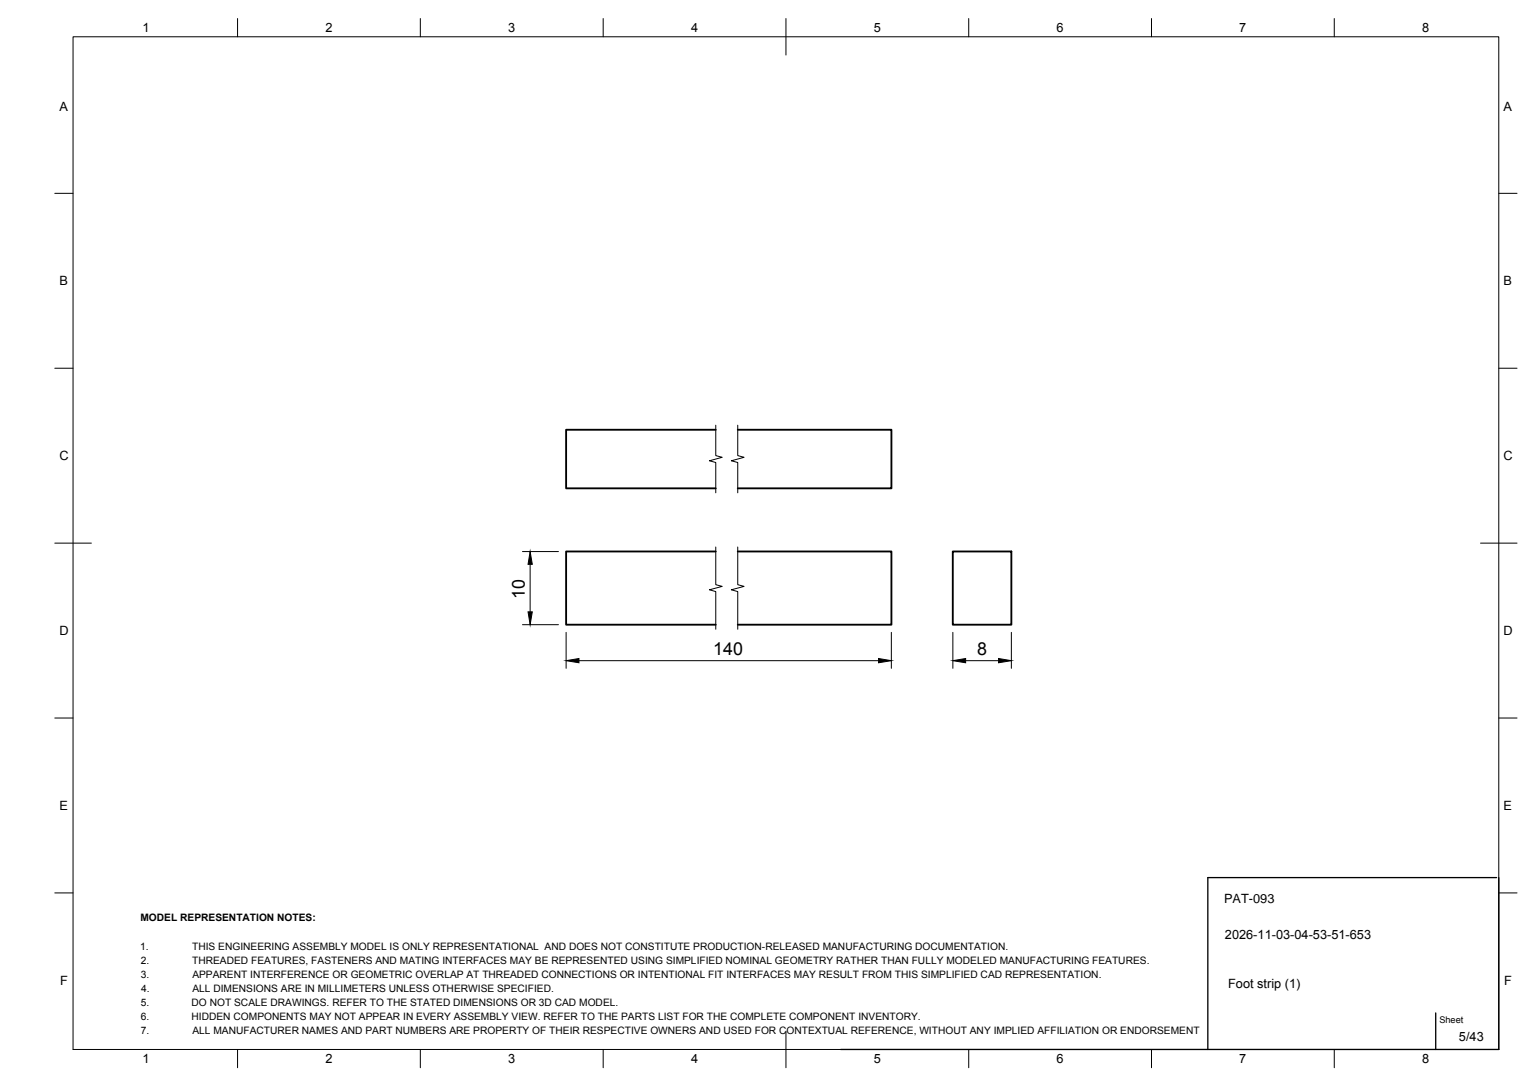
ISO-10303-21;
HEADER;
/* Generated by software containing ST-Developer
 * from STEP Tools, Inc. (www.steptools.com) 
 */

FILE_DESCRIPTION(
/* description */ ('Self-centering screw clamp'),
/* implementation_level */ '2;1');

FILE_NAME(
/* name */ 'Foot strip (1).step',
/* time_stamp */ '2026-10-28T03:25:31-07:00',
/* author */ (''),
/* organization */ (''),
/* preprocessor_version */ 'ST-DEVELOPER v20.2',
/* originating_system */ 'Autodesk Translation Framework v15.17.0.0',
/* authorisation */ '');

FILE_SCHEMA (('AUTOMOTIVE_DESIGN { 1 0 10303 214 3 1 1 }'));
ENDSEC;

DATA;
#10=MECHANICAL_DESIGN_GEOMETRIC_PRESENTATION_REPRESENTATION('',(#626),#16799);
#544=SHAPE_REPRESENTATION_RELATIONSHIP('SRR','None',#17017,#585);
#585=ADVANCED_BREP_SHAPE_REPRESENTATION('',(#674),#16755);
#626=STYLED_ITEM('',(#17312),#674);
#674=MANIFOLD_SOLID_BREP('Body1',#9077);
#1026=PLANE('',#9630);
#1027=PLANE('',#9631);
#1028=PLANE('',#9632);
#1029=PLANE('',#9633);
#1030=PLANE('',#9634);
#1031=PLANE('',#9635);
#1297=FACE_OUTER_BOUND('',#1825,.T.);
#1298=FACE_OUTER_BOUND('',#1826,.T.);
#1299=FACE_OUTER_BOUND('',#1827,.T.);
#1300=FACE_OUTER_BOUND('',#1828,.T.);
#1301=FACE_OUTER_BOUND('',#1829,.T.);
#1302=FACE_OUTER_BOUND('',#1830,.T.);
#1825=EDGE_LOOP('',(#6223,#6224,#6225,#6226));
#1826=EDGE_LOOP('',(#6227,#6228,#6229,#6230));
#1827=EDGE_LOOP('',(#6231,#6232,#6233,#6234));
#1828=EDGE_LOOP('',(#6235,#6236,#6237,#6238));
#1829=EDGE_LOOP('',(#6239,#6240,#6241,#6242));
#1830=EDGE_LOOP('',(#6243,#6244,#6245,#6246));
#2613=LINE('',#13807,#3186);
#2614=LINE('',#13809,#3187);
#2615=LINE('',#13811,#3188);
#2616=LINE('',#13812,#3189);
#2617=LINE('',#13815,#3190);
#2618=LINE('',#13817,#3191);
#2619=LINE('',#13818,#3192);
#2620=LINE('',#13821,#3193);
#2621=LINE('',#13823,#3194);
#2622=LINE('',#13824,#3195);
#2623=LINE('',#13826,#3196);
#2624=LINE('',#13827,#3197);
#3186=VECTOR('',#10896,1.);
#3187=VECTOR('',#10897,1.);
#3188=VECTOR('',#10898,1.);
#3189=VECTOR('',#10899,1.);
#3190=VECTOR('',#10902,1.);
#3191=VECTOR('',#10903,1.);
#3192=VECTOR('',#10904,1.);
#3193=VECTOR('',#10907,1.);
#3194=VECTOR('',#10908,1.);
#3195=VECTOR('',#10909,1.);
#3196=VECTOR('',#10912,1.);
#3197=VECTOR('',#10913,1.);
#4273=VERTEX_POINT('',#13805);
#4274=VERTEX_POINT('',#13806);
#4275=VERTEX_POINT('',#13808);
#4276=VERTEX_POINT('',#13810);
#4277=VERTEX_POINT('',#13814);
#4278=VERTEX_POINT('',#13816);
#4279=VERTEX_POINT('',#13820);
#4280=VERTEX_POINT('',#13822);
#5036=EDGE_CURVE('',#4273,#4274,#2613,.T.);
#5037=EDGE_CURVE('',#4274,#4275,#2614,.T.);
#5038=EDGE_CURVE('',#4276,#4275,#2615,.T.);
#5039=EDGE_CURVE('',#4273,#4276,#2616,.T.);
#5040=EDGE_CURVE('',#4277,#4273,#2617,.T.);
#5041=EDGE_CURVE('',#4278,#4276,#2618,.T.);
#5042=EDGE_CURVE('',#4277,#4278,#2619,.T.);
#5043=EDGE_CURVE('',#4279,#4277,#2620,.T.);
#5044=EDGE_CURVE('',#4280,#4278,#2621,.T.);
#5045=EDGE_CURVE('',#4279,#4280,#2622,.T.);
#5046=EDGE_CURVE('',#4274,#4279,#2623,.T.);
#5047=EDGE_CURVE('',#4275,#4280,#2624,.T.);
#6223=ORIENTED_EDGE('',*,*,#5036,.T.);
#6224=ORIENTED_EDGE('',*,*,#5037,.T.);
#6225=ORIENTED_EDGE('',*,*,#5038,.F.);
#6226=ORIENTED_EDGE('',*,*,#5039,.F.);
#6227=ORIENTED_EDGE('',*,*,#5040,.T.);
#6228=ORIENTED_EDGE('',*,*,#5039,.T.);
#6229=ORIENTED_EDGE('',*,*,#5041,.F.);
#6230=ORIENTED_EDGE('',*,*,#5042,.F.);
#6231=ORIENTED_EDGE('',*,*,#5043,.T.);
#6232=ORIENTED_EDGE('',*,*,#5042,.T.);
#6233=ORIENTED_EDGE('',*,*,#5044,.F.);
#6234=ORIENTED_EDGE('',*,*,#5045,.F.);
#6235=ORIENTED_EDGE('',*,*,#5046,.T.);
#6236=ORIENTED_EDGE('',*,*,#5045,.T.);
#6237=ORIENTED_EDGE('',*,*,#5047,.F.);
#6238=ORIENTED_EDGE('',*,*,#5037,.F.);
#6239=ORIENTED_EDGE('',*,*,#5047,.T.);
#6240=ORIENTED_EDGE('',*,*,#5044,.T.);
#6241=ORIENTED_EDGE('',*,*,#5041,.T.);
#6242=ORIENTED_EDGE('',*,*,#5038,.T.);
#6243=ORIENTED_EDGE('',*,*,#5046,.F.);
#6244=ORIENTED_EDGE('',*,*,#5036,.F.);
#6245=ORIENTED_EDGE('',*,*,#5040,.F.);
#6246=ORIENTED_EDGE('',*,*,#5043,.F.);
#8595=ADVANCED_FACE('',(#1297),#1026,.T.);
#8596=ADVANCED_FACE('',(#1298),#1027,.T.);
#8597=ADVANCED_FACE('',(#1299),#1028,.T.);
#8598=ADVANCED_FACE('',(#1300),#1029,.T.);
#8599=ADVANCED_FACE('',(#1301),#1030,.T.);
#8600=ADVANCED_FACE('',(#1302),#1031,.F.);
#9077=CLOSED_SHELL('',(#8595,#8596,#8597,#8598,#8599,#8600));
#9629=AXIS2_PLACEMENT_3D('',#13803,#10892,#10893);
#9630=AXIS2_PLACEMENT_3D('',#13804,#10894,#10895);
#9631=AXIS2_PLACEMENT_3D('',#13813,#10900,#10901);
#9632=AXIS2_PLACEMENT_3D('',#13819,#10905,#10906);
#9633=AXIS2_PLACEMENT_3D('',#13825,#10910,#10911);
#9634=AXIS2_PLACEMENT_3D('',#13828,#10914,#10915);
#9635=AXIS2_PLACEMENT_3D('',#13829,#10916,#10917);
#10892=DIRECTION('axis',(0.,0.,1.));
#10893=DIRECTION('refdir',(1.,0.,0.));
#10894=DIRECTION('center_axis',(0.,1.,0.));
#10895=DIRECTION('ref_axis',(-1.,0.,0.));
#10896=DIRECTION('',(-1.,0.,0.));
#10897=DIRECTION('',(0.,0.,1.));
#10898=DIRECTION('',(-1.,0.,0.));
#10899=DIRECTION('',(0.,0.,1.));
#10900=DIRECTION('center_axis',(1.,0.,0.));
#10901=DIRECTION('ref_axis',(0.,1.,0.));
#10902=DIRECTION('',(0.,1.,0.));
#10903=DIRECTION('',(0.,1.,0.));
#10904=DIRECTION('',(0.,0.,1.));
#10905=DIRECTION('center_axis',(0.,-1.,0.));
#10906=DIRECTION('ref_axis',(1.,0.,0.));
#10907=DIRECTION('',(1.,0.,0.));
#10908=DIRECTION('',(1.,0.,0.));
#10909=DIRECTION('',(0.,0.,1.));
#10910=DIRECTION('center_axis',(-1.,0.,0.));
#10911=DIRECTION('ref_axis',(0.,-1.,0.));
#10912=DIRECTION('',(0.,-1.,0.));
#10913=DIRECTION('',(0.,-1.,0.));
#10914=DIRECTION('center_axis',(0.,0.,1.));
#10915=DIRECTION('ref_axis',(1.,0.,0.));
#10916=DIRECTION('center_axis',(0.,0.,1.));
#10917=DIRECTION('ref_axis',(1.,0.,0.));
#13803=CARTESIAN_POINT('',(0.,0.,0.));
#13804=CARTESIAN_POINT('Origin',(16.,7.,-0.8));
#13805=CARTESIAN_POINT('',(16.,7.,-0.8));
#13806=CARTESIAN_POINT('',(15.,7.,-0.8));
#13807=CARTESIAN_POINT('',(16.,7.,-0.8));
#13808=CARTESIAN_POINT('',(15.,7.,0.));
#13809=CARTESIAN_POINT('',(15.,7.,-0.8));
#13810=CARTESIAN_POINT('',(16.,7.,0.));
#13811=CARTESIAN_POINT('',(16.,7.,0.));
#13812=CARTESIAN_POINT('',(16.,7.,-0.8));
#13813=CARTESIAN_POINT('Origin',(16.,-7.,-0.8));
#13814=CARTESIAN_POINT('',(16.,-7.,-0.8));
#13815=CARTESIAN_POINT('',(16.,-7.,-0.8));
#13816=CARTESIAN_POINT('',(16.,-7.,0.));
#13817=CARTESIAN_POINT('',(16.,-7.,0.));
#13818=CARTESIAN_POINT('',(16.,-7.,-0.8));
#13819=CARTESIAN_POINT('Origin',(15.,-7.,-0.8));
#13820=CARTESIAN_POINT('',(15.,-7.,-0.8));
#13821=CARTESIAN_POINT('',(15.,-7.,-0.8));
#13822=CARTESIAN_POINT('',(15.,-7.,0.));
#13823=CARTESIAN_POINT('',(15.,-7.,0.));
#13824=CARTESIAN_POINT('',(15.,-7.,-0.8));
#13825=CARTESIAN_POINT('Origin',(15.,7.,-0.8));
#13826=CARTESIAN_POINT('',(15.,7.,-0.8));
#13827=CARTESIAN_POINT('',(15.,7.,0.));
#13828=CARTESIAN_POINT('Origin',(15.5,0.,0.));
#13829=CARTESIAN_POINT('Origin',(15.5,0.,-0.8));
#16706=UNCERTAINTY_MEASURE_WITH_UNIT(LENGTH_MEASURE(0.001),#16800,
'DISTANCE_ACCURACY_VALUE',
'Maximum model space distance between geometric entities at asserted c
onnectivities');
#16750=UNCERTAINTY_MEASURE_WITH_UNIT(LENGTH_MEASURE(0.001),#16800,
'DISTANCE_ACCURACY_VALUE',
'Maximum model space distance between geometric entities at asserted c
onnectivities');
#16755=(
GEOMETRIC_REPRESENTATION_CONTEXT(3)
GLOBAL_UNCERTAINTY_ASSIGNED_CONTEXT((#16706))
GLOBAL_UNIT_ASSIGNED_CONTEXT((#16800,#16802,#16803))
REPRESENTATION_CONTEXT('','3D')
);
#16799=(
GEOMETRIC_REPRESENTATION_CONTEXT(3)
GLOBAL_UNCERTAINTY_ASSIGNED_CONTEXT((#16750))
GLOBAL_UNIT_ASSIGNED_CONTEXT((#16800,#16802,#16803))
REPRESENTATION_CONTEXT('','3D')
);
#16800=(
LENGTH_UNIT()
NAMED_UNIT(*)
SI_UNIT(.CENTI.,.METRE.)
);
#16802=(
NAMED_UNIT(*)
PLANE_ANGLE_UNIT()
SI_UNIT($,.RADIAN.)
);
#16803=(
NAMED_UNIT(*)
SI_UNIT($,.STERADIAN.)
SOLID_ANGLE_UNIT()
);
#16808=SHAPE_DEFINITION_REPRESENTATION(#16856,#17017);
#16856=PRODUCT_DEFINITION_SHAPE('',$,#17066);
#17017=SHAPE_REPRESENTATION('',(#9629),#16755);
#17061=PRODUCT_DEFINITION_CONTEXT('part definition',#17207,'design');
#17066=PRODUCT_DEFINITION('Foot strip (1)','Foot strip (1)',#17114,#17061);
#17114=PRODUCT_DEFINITION_FORMATION('',$,#17213);
#17207=APPLICATION_CONTEXT(
'Core Data for Automotive Mechanical Design Process');
#17208=PRODUCT_CONTEXT('part definition',#17207,'mechanical');
#17213=PRODUCT('Foot strip (1)','Foot strip (1)','Foot strip (1)',(#17208));
#17306=COLOUR_RGB('Light Blue',0.38,0.62,0.78);
#17307=FILL_AREA_STYLE_COLOUR('',#17306);
#17308=FILL_AREA_STYLE('',(#17307));
#17309=SURFACE_STYLE_FILL_AREA(#17308);
#17310=SURFACE_SIDE_STYLE('',(#17309));
#17311=SURFACE_STYLE_USAGE(.BOTH.,#17310);
#17312=PRESENTATION_STYLE_ASSIGNMENT((#17311));
ENDSEC;
END-ISO-10303-21;
